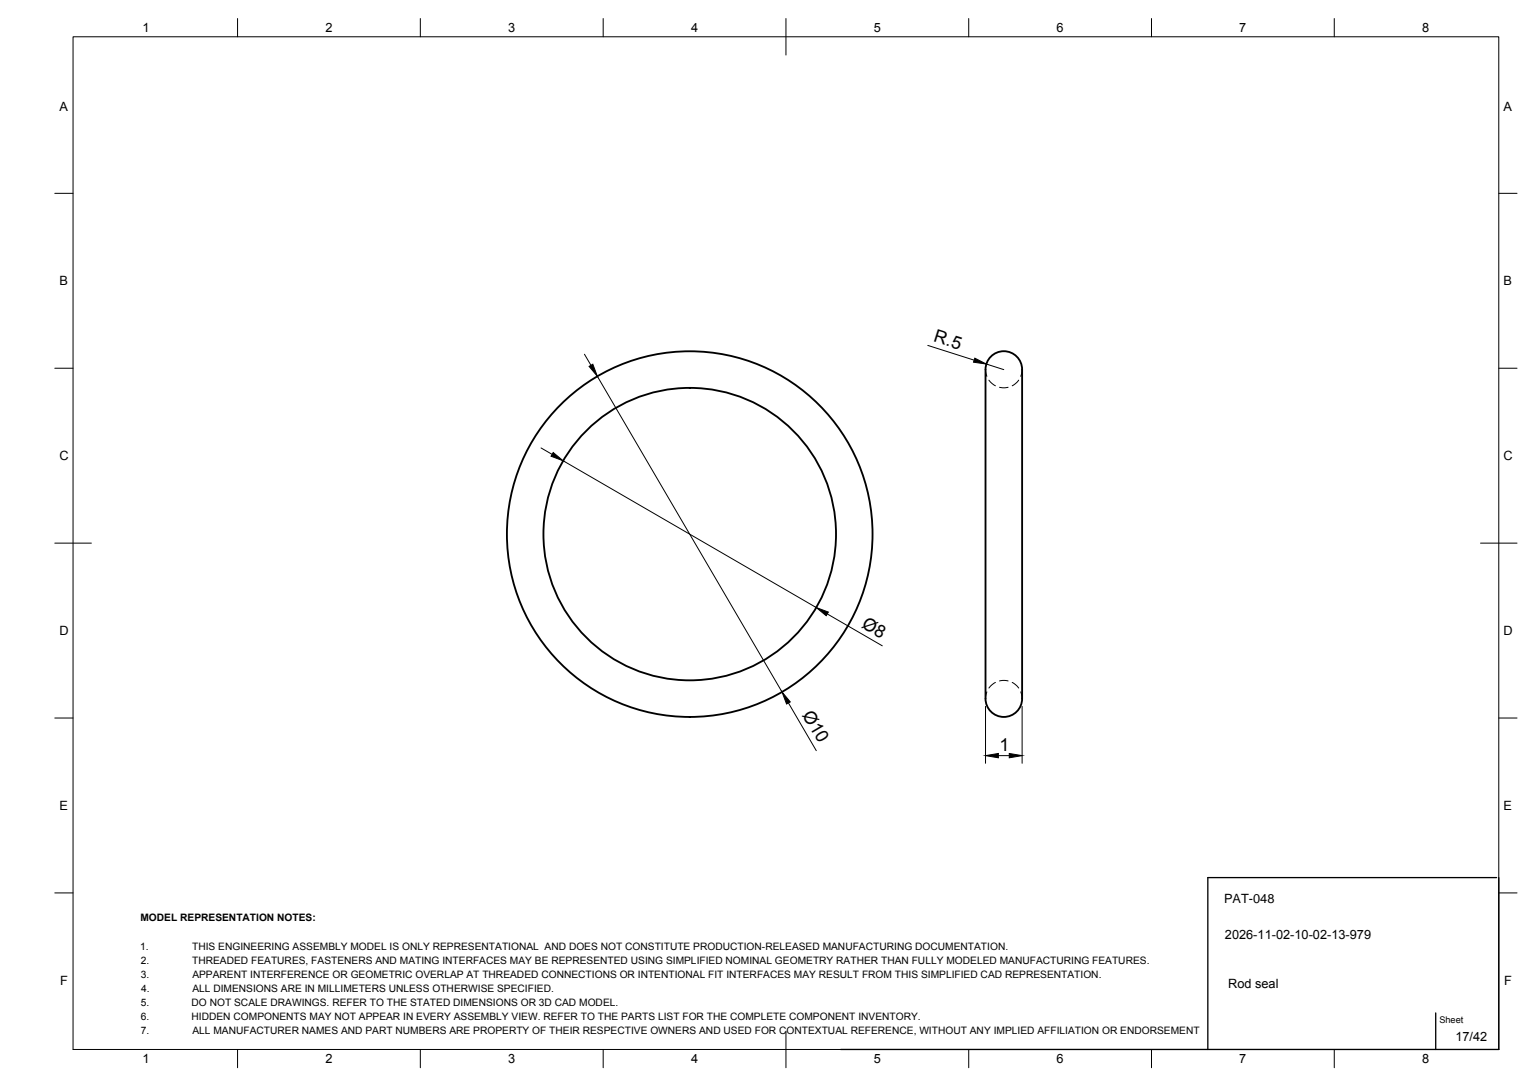
ISO-10303-21;
HEADER;
/* Generated by software containing ST-Developer
 * from STEP Tools, Inc. (www.steptools.com) 
 */

FILE_DESCRIPTION(
/* description */ ('Guided pneumatic stop gate'),
/* implementation_level */ '2;1');

FILE_NAME(
/* name */ 'Rod seal.step',
/* time_stamp */ '2026-10-27T21:43:45-07:00',
/* author */ (''),
/* organization */ (''),
/* preprocessor_version */ 'ST-DEVELOPER v20.2',
/* originating_system */ 'Autodesk Translation Framework v15.17.0.0',
/* authorisation */ '');

FILE_SCHEMA (('AUTOMOTIVE_DESIGN { 1 0 10303 214 3 1 1 }'));
ENDSEC;

DATA;
#10=MECHANICAL_DESIGN_GEOMETRIC_PRESENTATION_REPRESENTATION('',(#550),#14392);
#44=TOROIDAL_SURFACE('',#8789,0.45,0.05);
#466=SHAPE_REPRESENTATION_RELATIONSHIP('SRR','None',#14601,#508);
#508=ADVANCED_BREP_SHAPE_REPRESENTATION('',(#591),#14363);
#550=STYLED_ITEM('',(#14898),#591);
#591=MANIFOLD_SOLID_BREP('Body1',#7891);
#1330=FACE_OUTER_BOUND('',#1885,.T.);
#1885=EDGE_LOOP('',(#6146,#6147,#6148,#6149));
#3526=CIRCLE('',#8790,0.05);
#3527=CIRCLE('',#8791,0.4);
#4000=VERTEX_POINT('',#12832);
#4771=EDGE_CURVE('',#4000,#4000,#3526,.T.);
#4772=EDGE_CURVE('',#4000,#4000,#3527,.T.);
#6146=ORIENTED_EDGE('',*,*,#4771,.F.);
#6147=ORIENTED_EDGE('',*,*,#4772,.T.);
#6148=ORIENTED_EDGE('',*,*,#4771,.T.);
#6149=ORIENTED_EDGE('',*,*,#4772,.F.);
#7612=ADVANCED_FACE('',(#1330),#44,.T.);
#7891=CLOSED_SHELL('',(#7612));
#8788=AXIS2_PLACEMENT_3D('',#12830,#10432,#10433);
#8789=AXIS2_PLACEMENT_3D('',#12831,#10434,#10435);
#8790=AXIS2_PLACEMENT_3D('',#12833,#10436,#10437);
#8791=AXIS2_PLACEMENT_3D('',#12834,#10438,#10439);
#10432=DIRECTION('axis',(0.,0.,1.));
#10433=DIRECTION('refdir',(1.,0.,0.));
#10434=DIRECTION('center_axis',(0.,-1.,0.));
#10435=DIRECTION('ref_axis',(0.,0.,-1.));
#10436=DIRECTION('center_axis',(-1.,0.,-1.22464679914735E-16));
#10437=DIRECTION('ref_axis',(-1.22464679914735E-16,0.,1.));
#10438=DIRECTION('center_axis',(0.,1.,0.));
#10439=DIRECTION('ref_axis',(0.,0.,-1.));
#12830=CARTESIAN_POINT('',(0.,0.,0.));
#12831=CARTESIAN_POINT('Origin',(0.,0.2,4.5));
#12832=CARTESIAN_POINT('',(-4.89858719658941E-17,0.2,4.9));
#12833=CARTESIAN_POINT('Origin',(-5.51091059616309E-17,0.2,4.95));
#12834=CARTESIAN_POINT('Origin',(0.,0.2,4.5));
#14315=UNCERTAINTY_MEASURE_WITH_UNIT(LENGTH_MEASURE(0.001),#14393,
'DISTANCE_ACCURACY_VALUE',
'Maximum model space distance between geometric entities at asserted c
onnectivities');
#14344=UNCERTAINTY_MEASURE_WITH_UNIT(LENGTH_MEASURE(0.001),#14393,
'DISTANCE_ACCURACY_VALUE',
'Maximum model space distance between geometric entities at asserted c
onnectivities');
#14363=(
GEOMETRIC_REPRESENTATION_CONTEXT(3)
GLOBAL_UNCERTAINTY_ASSIGNED_CONTEXT((#14315))
GLOBAL_UNIT_ASSIGNED_CONTEXT((#14393,#14395,#14396))
REPRESENTATION_CONTEXT('','3D')
);
#14392=(
GEOMETRIC_REPRESENTATION_CONTEXT(3)
GLOBAL_UNCERTAINTY_ASSIGNED_CONTEXT((#14344))
GLOBAL_UNIT_ASSIGNED_CONTEXT((#14393,#14395,#14396))
REPRESENTATION_CONTEXT('','3D')
);
#14393=(
LENGTH_UNIT()
NAMED_UNIT(*)
SI_UNIT(.CENTI.,.METRE.)
);
#14395=(
NAMED_UNIT(*)
PLANE_ANGLE_UNIT()
SI_UNIT($,.RADIAN.)
);
#14396=(
NAMED_UNIT(*)
SI_UNIT($,.STERADIAN.)
SOLID_ANGLE_UNIT()
);
#14415=SHAPE_DEFINITION_REPRESENTATION(#14464,#14601);
#14464=PRODUCT_DEFINITION_SHAPE('',$,#14649);
#14601=SHAPE_REPRESENTATION('',(#8788),#14363);
#14630=PRODUCT_DEFINITION_CONTEXT('part definition',#14773,'design');
#14649=PRODUCT_DEFINITION('Rod seal','Rod seal',#14696,#14630);
#14696=PRODUCT_DEFINITION_FORMATION('',$,#14793);
#14773=APPLICATION_CONTEXT(
'Core Data for Automotive Mechanical Design Process');
#14774=PRODUCT_CONTEXT('part definition',#14773,'mechanical');
#14793=PRODUCT('Rod seal','Rod seal','Rod seal',(#14774));
#14892=COLOUR_RGB('Black',0.12,0.14,0.17);
#14893=FILL_AREA_STYLE_COLOUR('',#14892);
#14894=FILL_AREA_STYLE('',(#14893));
#14895=SURFACE_STYLE_FILL_AREA(#14894);
#14896=SURFACE_SIDE_STYLE('',(#14895));
#14897=SURFACE_STYLE_USAGE(.BOTH.,#14896);
#14898=PRESENTATION_STYLE_ASSIGNMENT((#14897));
ENDSEC;
END-ISO-10303-21;
